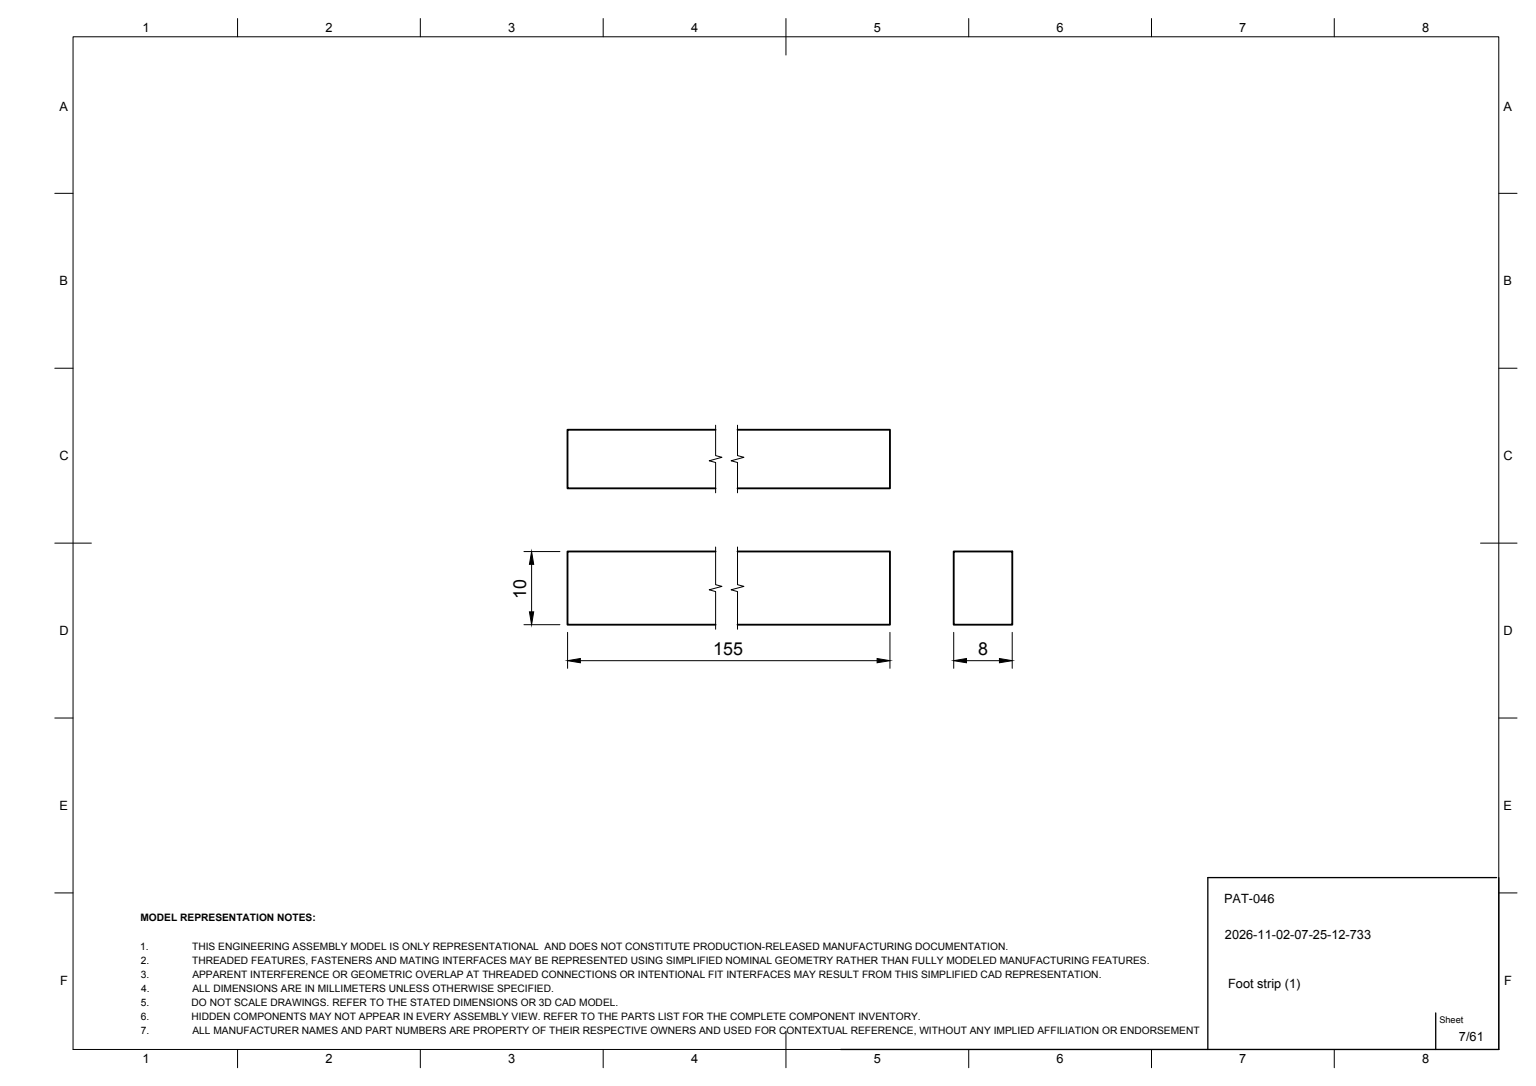
ISO-10303-21;
HEADER;
/* Generated by software containing ST-Developer
 * from STEP Tools, Inc. (www.steptools.com) 
 */

FILE_DESCRIPTION(
/* description */ ('Gear mesh backlash fixture'),
/* implementation_level */ '2;1');

FILE_NAME(
/* name */ 'Foot strip (1).step',
/* time_stamp */ '2026-10-28T03:26:00-07:00',
/* author */ (''),
/* organization */ (''),
/* preprocessor_version */ 'ST-DEVELOPER v20.2',
/* originating_system */ 'Autodesk Translation Framework v15.17.0.0',
/* authorisation */ '');

FILE_SCHEMA (('AUTOMOTIVE_DESIGN { 1 0 10303 214 3 1 1 }'));
ENDSEC;

DATA;
#10=MECHANICAL_DESIGN_GEOMETRIC_PRESENTATION_REPRESENTATION('',(#1018),#57900);
#918=SHAPE_REPRESENTATION_RELATIONSHIP('SRR','None',#58113,#968);
#968=ADVANCED_BREP_SHAPE_REPRESENTATION('',(#1083),#57846);
#1018=STYLED_ITEM('',(#58451),#1083);
#1083=MANIFOLD_SOLID_BREP('Body1',#13578);
#1342=PLANE('',#14248);
#1343=PLANE('',#14249);
#1344=PLANE('',#14250);
#1345=PLANE('',#14251);
#1346=PLANE('',#14252);
#1347=PLANE('',#14253);
#1718=FACE_OUTER_BOUND('',#2507,.T.);
#1719=FACE_OUTER_BOUND('',#2508,.T.);
#1720=FACE_OUTER_BOUND('',#2509,.T.);
#1721=FACE_OUTER_BOUND('',#2510,.T.);
#1722=FACE_OUTER_BOUND('',#2511,.T.);
#1723=FACE_OUTER_BOUND('',#2512,.T.);
#2507=EDGE_LOOP('',(#8999,#9000,#9001,#9002));
#2508=EDGE_LOOP('',(#9003,#9004,#9005,#9006));
#2509=EDGE_LOOP('',(#9007,#9008,#9009,#9010));
#2510=EDGE_LOOP('',(#9011,#9012,#9013,#9014));
#2511=EDGE_LOOP('',(#9015,#9016,#9017,#9018));
#2512=EDGE_LOOP('',(#9019,#9020,#9021,#9022));
#3447=LINE('',#19365,#4336);
#3448=LINE('',#19367,#4337);
#3449=LINE('',#19369,#4338);
#3450=LINE('',#19370,#4339);
#3451=LINE('',#19373,#4340);
#3452=LINE('',#19375,#4341);
#3453=LINE('',#19376,#4342);
#3454=LINE('',#19379,#4343);
#3455=LINE('',#19381,#4344);
#3456=LINE('',#19382,#4345);
#3457=LINE('',#19384,#4346);
#3458=LINE('',#19385,#4347);
#4336=VECTOR('',#15722,1.);
#4337=VECTOR('',#15723,1.);
#4338=VECTOR('',#15724,1.);
#4339=VECTOR('',#15725,1.);
#4340=VECTOR('',#15728,1.);
#4341=VECTOR('',#15729,1.);
#4342=VECTOR('',#15730,1.);
#4343=VECTOR('',#15733,1.);
#4344=VECTOR('',#15734,1.);
#4345=VECTOR('',#15735,1.);
#4346=VECTOR('',#15738,1.);
#4347=VECTOR('',#15739,1.);
#5821=VERTEX_POINT('',#19363);
#5822=VERTEX_POINT('',#19364);
#5823=VERTEX_POINT('',#19366);
#5824=VERTEX_POINT('',#19368);
#5825=VERTEX_POINT('',#19372);
#5826=VERTEX_POINT('',#19374);
#5827=VERTEX_POINT('',#19378);
#5828=VERTEX_POINT('',#19380);
#7086=EDGE_CURVE('',#5821,#5822,#3447,.T.);
#7087=EDGE_CURVE('',#5822,#5823,#3448,.T.);
#7088=EDGE_CURVE('',#5824,#5823,#3449,.T.);
#7089=EDGE_CURVE('',#5821,#5824,#3450,.T.);
#7090=EDGE_CURVE('',#5825,#5821,#3451,.T.);
#7091=EDGE_CURVE('',#5826,#5824,#3452,.T.);
#7092=EDGE_CURVE('',#5825,#5826,#3453,.T.);
#7093=EDGE_CURVE('',#5827,#5825,#3454,.T.);
#7094=EDGE_CURVE('',#5828,#5826,#3455,.T.);
#7095=EDGE_CURVE('',#5827,#5828,#3456,.T.);
#7096=EDGE_CURVE('',#5822,#5827,#3457,.T.);
#7097=EDGE_CURVE('',#5823,#5828,#3458,.T.);
#8999=ORIENTED_EDGE('',*,*,#7086,.T.);
#9000=ORIENTED_EDGE('',*,*,#7087,.T.);
#9001=ORIENTED_EDGE('',*,*,#7088,.F.);
#9002=ORIENTED_EDGE('',*,*,#7089,.F.);
#9003=ORIENTED_EDGE('',*,*,#7090,.T.);
#9004=ORIENTED_EDGE('',*,*,#7089,.T.);
#9005=ORIENTED_EDGE('',*,*,#7091,.F.);
#9006=ORIENTED_EDGE('',*,*,#7092,.F.);
#9007=ORIENTED_EDGE('',*,*,#7093,.T.);
#9008=ORIENTED_EDGE('',*,*,#7092,.T.);
#9009=ORIENTED_EDGE('',*,*,#7094,.F.);
#9010=ORIENTED_EDGE('',*,*,#7095,.F.);
#9011=ORIENTED_EDGE('',*,*,#7096,.T.);
#9012=ORIENTED_EDGE('',*,*,#7095,.T.);
#9013=ORIENTED_EDGE('',*,*,#7097,.F.);
#9014=ORIENTED_EDGE('',*,*,#7087,.F.);
#9015=ORIENTED_EDGE('',*,*,#7097,.T.);
#9016=ORIENTED_EDGE('',*,*,#7094,.T.);
#9017=ORIENTED_EDGE('',*,*,#7091,.T.);
#9018=ORIENTED_EDGE('',*,*,#7088,.T.);
#9019=ORIENTED_EDGE('',*,*,#7096,.F.);
#9020=ORIENTED_EDGE('',*,*,#7086,.F.);
#9021=ORIENTED_EDGE('',*,*,#7090,.F.);
#9022=ORIENTED_EDGE('',*,*,#7093,.F.);
#12835=ADVANCED_FACE('',(#1718),#1342,.T.);
#12836=ADVANCED_FACE('',(#1719),#1343,.T.);
#12837=ADVANCED_FACE('',(#1720),#1344,.T.);
#12838=ADVANCED_FACE('',(#1721),#1345,.T.);
#12839=ADVANCED_FACE('',(#1722),#1346,.T.);
#12840=ADVANCED_FACE('',(#1723),#1347,.F.);
#13578=CLOSED_SHELL('',(#12835,#12836,#12837,#12838,#12839,#12840));
#14247=AXIS2_PLACEMENT_3D('',#19361,#15718,#15719);
#14248=AXIS2_PLACEMENT_3D('',#19362,#15720,#15721);
#14249=AXIS2_PLACEMENT_3D('',#19371,#15726,#15727);
#14250=AXIS2_PLACEMENT_3D('',#19377,#15731,#15732);
#14251=AXIS2_PLACEMENT_3D('',#19383,#15736,#15737);
#14252=AXIS2_PLACEMENT_3D('',#19386,#15740,#15741);
#14253=AXIS2_PLACEMENT_3D('',#19387,#15742,#15743);
#15718=DIRECTION('axis',(0.,0.,1.));
#15719=DIRECTION('refdir',(1.,0.,0.));
#15720=DIRECTION('center_axis',(0.,1.,0.));
#15721=DIRECTION('ref_axis',(-1.,0.,0.));
#15722=DIRECTION('',(-1.,0.,0.));
#15723=DIRECTION('',(0.,0.,1.));
#15724=DIRECTION('',(-1.,0.,0.));
#15725=DIRECTION('',(0.,0.,1.));
#15726=DIRECTION('center_axis',(1.,0.,0.));
#15727=DIRECTION('ref_axis',(0.,1.,0.));
#15728=DIRECTION('',(0.,1.,0.));
#15729=DIRECTION('',(0.,1.,0.));
#15730=DIRECTION('',(0.,0.,1.));
#15731=DIRECTION('center_axis',(0.,-1.,0.));
#15732=DIRECTION('ref_axis',(1.,0.,0.));
#15733=DIRECTION('',(1.,0.,0.));
#15734=DIRECTION('',(1.,0.,0.));
#15735=DIRECTION('',(0.,0.,1.));
#15736=DIRECTION('center_axis',(-1.,0.,0.));
#15737=DIRECTION('ref_axis',(0.,-1.,0.));
#15738=DIRECTION('',(0.,-1.,0.));
#15739=DIRECTION('',(0.,-1.,0.));
#15740=DIRECTION('center_axis',(0.,0.,1.));
#15741=DIRECTION('ref_axis',(1.,0.,0.));
#15742=DIRECTION('center_axis',(0.,0.,1.));
#15743=DIRECTION('ref_axis',(1.,0.,0.));
#19361=CARTESIAN_POINT('',(0.,0.,0.));
#19362=CARTESIAN_POINT('Origin',(21.,11.5,-1.8));
#19363=CARTESIAN_POINT('',(21.,11.5,-1.8));
#19364=CARTESIAN_POINT('',(20.,11.5,-1.8));
#19365=CARTESIAN_POINT('',(21.,11.5,-1.8));
#19366=CARTESIAN_POINT('',(20.,11.5,-1.));
#19367=CARTESIAN_POINT('',(20.,11.5,-1.8));
#19368=CARTESIAN_POINT('',(21.,11.5,-1.));
#19369=CARTESIAN_POINT('',(21.,11.5,-1.));
#19370=CARTESIAN_POINT('',(21.,11.5,-1.8));
#19371=CARTESIAN_POINT('Origin',(21.,-4.,-1.8));
#19372=CARTESIAN_POINT('',(21.,-4.,-1.8));
#19373=CARTESIAN_POINT('',(21.,-4.,-1.8));
#19374=CARTESIAN_POINT('',(21.,-4.,-1.));
#19375=CARTESIAN_POINT('',(21.,-4.,-1.));
#19376=CARTESIAN_POINT('',(21.,-4.,-1.8));
#19377=CARTESIAN_POINT('Origin',(20.,-4.,-1.8));
#19378=CARTESIAN_POINT('',(20.,-4.,-1.8));
#19379=CARTESIAN_POINT('',(20.,-4.,-1.8));
#19380=CARTESIAN_POINT('',(20.,-4.,-1.));
#19381=CARTESIAN_POINT('',(20.,-4.,-1.));
#19382=CARTESIAN_POINT('',(20.,-4.,-1.8));
#19383=CARTESIAN_POINT('Origin',(20.,11.5,-1.8));
#19384=CARTESIAN_POINT('',(20.,11.5,-1.8));
#19385=CARTESIAN_POINT('',(20.,11.5,-1.));
#19386=CARTESIAN_POINT('Origin',(20.5,3.75,-1.));
#19387=CARTESIAN_POINT('Origin',(20.5,3.75,-1.8));
#57787=UNCERTAINTY_MEASURE_WITH_UNIT(LENGTH_MEASURE(0.001),#57901,
'DISTANCE_ACCURACY_VALUE',
'Maximum model space distance between geometric entities at asserted c
onnectivities');
#57841=UNCERTAINTY_MEASURE_WITH_UNIT(LENGTH_MEASURE(0.001),#57901,
'DISTANCE_ACCURACY_VALUE',
'Maximum model space distance between geometric entities at asserted c
onnectivities');
#57846=(
GEOMETRIC_REPRESENTATION_CONTEXT(3)
GLOBAL_UNCERTAINTY_ASSIGNED_CONTEXT((#57787))
GLOBAL_UNIT_ASSIGNED_CONTEXT((#57901,#57903,#57904))
REPRESENTATION_CONTEXT('','3D')
);
#57900=(
GEOMETRIC_REPRESENTATION_CONTEXT(3)
GLOBAL_UNCERTAINTY_ASSIGNED_CONTEXT((#57841))
GLOBAL_UNIT_ASSIGNED_CONTEXT((#57901,#57903,#57904))
REPRESENTATION_CONTEXT('','3D')
);
#57901=(
LENGTH_UNIT()
NAMED_UNIT(*)
SI_UNIT(.CENTI.,.METRE.)
);
#57903=(
NAMED_UNIT(*)
PLANE_ANGLE_UNIT()
SI_UNIT($,.RADIAN.)
);
#57904=(
NAMED_UNIT(*)
SI_UNIT($,.STERADIAN.)
SOLID_ANGLE_UNIT()
);
#57909=SHAPE_DEFINITION_REPRESENTATION(#57967,#58113);
#57967=PRODUCT_DEFINITION_SHAPE('',$,#58172);
#58113=SHAPE_REPRESENTATION('',(#14247),#57846);
#58167=PRODUCT_DEFINITION_CONTEXT('part definition',#58343,'design');
#58172=PRODUCT_DEFINITION('Foot strip (1)','Foot strip (1)',#58230,#58167);
#58230=PRODUCT_DEFINITION_FORMATION('',$,#58349);
#58343=APPLICATION_CONTEXT(
'Core Data for Automotive Mechanical Design Process');
#58344=PRODUCT_CONTEXT('part definition',#58343,'mechanical');
#58349=PRODUCT('Foot strip (1)','Foot strip (1)','Foot strip (1)',(#58344));
#58445=COLOUR_RGB('Light Blue',0.38,0.62,0.78);
#58446=FILL_AREA_STYLE_COLOUR('',#58445);
#58447=FILL_AREA_STYLE('',(#58446));
#58448=SURFACE_STYLE_FILL_AREA(#58447);
#58449=SURFACE_SIDE_STYLE('',(#58448));
#58450=SURFACE_STYLE_USAGE(.BOTH.,#58449);
#58451=PRESENTATION_STYLE_ASSIGNMENT((#58450));
ENDSEC;
END-ISO-10303-21;
